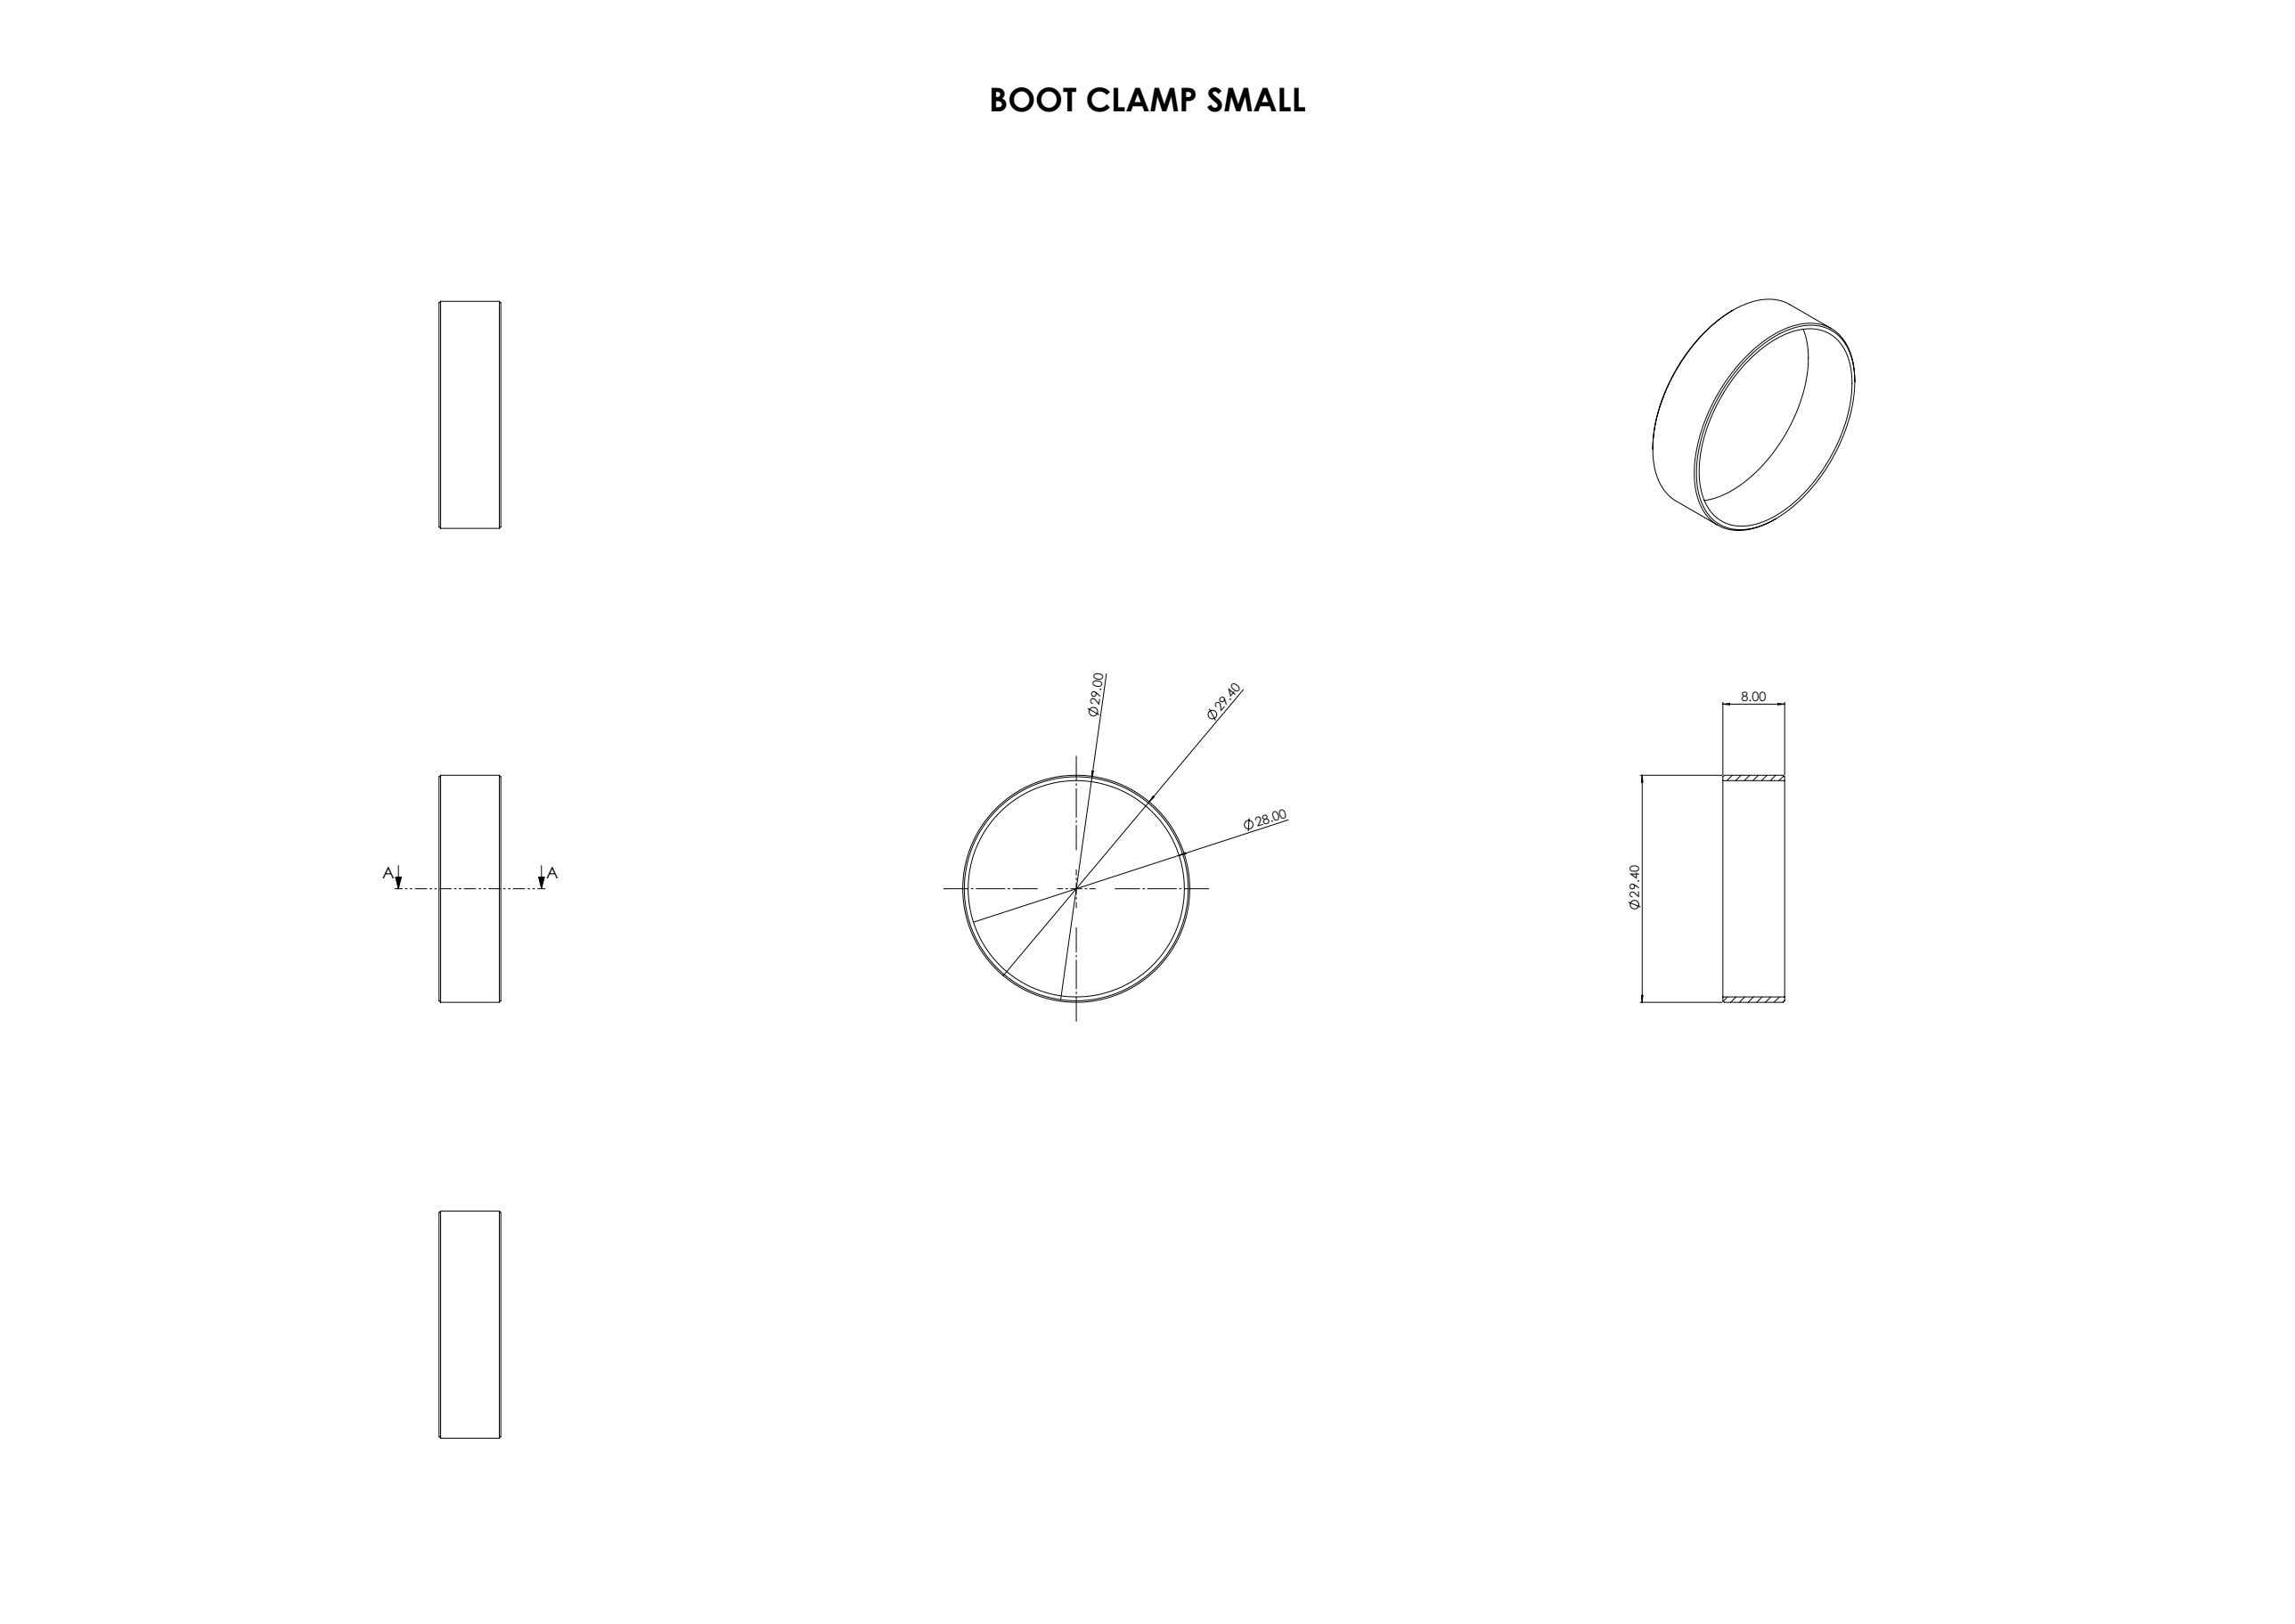
ISO-10303-21;
HEADER;
/* Generated by software containing ST-Developer
 * from STEP Tools, Inc. (www.steptools.com) 
 */

FILE_DESCRIPTION(
/* description */ (''),
/* implementation_level */ '2;1');

FILE_NAME(
/* name */ '09_Boot_Clamp_Small.step',
/* time_stamp */ '2026-10-11T12:57:03-07:00',
/* author */ (''),
/* organization */ (''),
/* preprocessor_version */ 'ST-DEVELOPER v20.2',
/* originating_system */ 'Autodesk Translation Framework v15.15.0.0',
/* authorisation */ '');

FILE_SCHEMA (('AUTOMOTIVE_DESIGN { 1 0 10303 214 3 1 1 }'));
ENDSEC;

DATA;
#10=MECHANICAL_DESIGN_GEOMETRIC_PRESENTATION_REPRESENTATION('',(#264),#90374);
#230=SHAPE_REPRESENTATION_RELATIONSHIP('SRR','None',#90449,#247);
#247=ADVANCED_BREP_SHAPE_REPRESENTATION('',(#281),#90365);
#264=STYLED_ITEM('',(#90673),#281);
#281=MANIFOLD_SOLID_BREP('Body1',#40353);
#691=CONICAL_SURFACE('',#43833,14.6,0.785398163397449);
#692=CONICAL_SURFACE('',#43838,14.6,0.785398163397448);
#1071=FACE_BOUND('',#6255,.T.);
#1072=FACE_BOUND('',#6258,.T.);
#1441=PLANE('',#43840);
#1442=PLANE('',#43844);
#3823=FACE_OUTER_BOUND('',#6251,.T.);
#3824=FACE_OUTER_BOUND('',#6252,.T.);
#3825=FACE_OUTER_BOUND('',#6253,.T.);
#3826=FACE_OUTER_BOUND('',#6254,.T.);
#3827=FACE_OUTER_BOUND('',#6256,.T.);
#3828=FACE_OUTER_BOUND('',#6257,.T.);
#6251=EDGE_LOOP('',(#33331,#33332,#33333,#33334));
#6252=EDGE_LOOP('',(#33335,#33336,#33337,#33338));
#6253=EDGE_LOOP('',(#33339,#33340,#33341,#33342));
#6254=EDGE_LOOP('',(#33343));
#6255=EDGE_LOOP('',(#33344));
#6256=EDGE_LOOP('',(#33345,#33346,#33347,#33348));
#6257=EDGE_LOOP('',(#33349));
#6258=EDGE_LOOP('',(#33350));
#8699=CIRCLE('',#43834,14.7);
#8700=CIRCLE('',#43835,14.5);
#8701=CIRCLE('',#43837,14.7);
#8702=CIRCLE('',#43839,14.5);
#8703=CIRCLE('',#43841,14.);
#8704=CIRCLE('',#43843,14.);
#11851=LINE('',#83003,#14345);
#11852=LINE('',#83008,#14346);
#11853=LINE('',#83012,#14347);
#11854=LINE('',#83018,#14348);
#14345=VECTOR('',#53359,14.6);
#14346=VECTOR('',#53366,14.7);
#14347=VECTOR('',#53371,14.6);
#14348=VECTOR('',#53378,14.);
#17794=VERTEX_POINT('',#83000);
#17795=VERTEX_POINT('',#83002);
#17796=VERTEX_POINT('',#83006);
#17797=VERTEX_POINT('',#83010);
#17798=VERTEX_POINT('',#83014);
#17799=VERTEX_POINT('',#83017);
#23177=EDGE_CURVE('',#17794,#17794,#8699,.T.);
#23178=EDGE_CURVE('',#17794,#17795,#11851,.T.);
#23179=EDGE_CURVE('',#17795,#17795,#8700,.T.);
#23180=EDGE_CURVE('',#17796,#17796,#8701,.T.);
#23181=EDGE_CURVE('',#17796,#17794,#11852,.T.);
#23182=EDGE_CURVE('',#17797,#17797,#8702,.T.);
#23183=EDGE_CURVE('',#17797,#17796,#11853,.T.);
#23184=EDGE_CURVE('',#17798,#17798,#8703,.T.);
#23185=EDGE_CURVE('',#17798,#17799,#11854,.T.);
#23186=EDGE_CURVE('',#17799,#17799,#8704,.T.);
#33331=ORIENTED_EDGE('',*,*,#23177,.F.);
#33332=ORIENTED_EDGE('',*,*,#23178,.T.);
#33333=ORIENTED_EDGE('',*,*,#23179,.T.);
#33334=ORIENTED_EDGE('',*,*,#23178,.F.);
#33335=ORIENTED_EDGE('',*,*,#23180,.F.);
#33336=ORIENTED_EDGE('',*,*,#23181,.T.);
#33337=ORIENTED_EDGE('',*,*,#23177,.T.);
#33338=ORIENTED_EDGE('',*,*,#23181,.F.);
#33339=ORIENTED_EDGE('',*,*,#23182,.F.);
#33340=ORIENTED_EDGE('',*,*,#23183,.T.);
#33341=ORIENTED_EDGE('',*,*,#23180,.T.);
#33342=ORIENTED_EDGE('',*,*,#23183,.F.);
#33343=ORIENTED_EDGE('',*,*,#23182,.T.);
#33344=ORIENTED_EDGE('',*,*,#23184,.F.);
#33345=ORIENTED_EDGE('',*,*,#23184,.T.);
#33346=ORIENTED_EDGE('',*,*,#23185,.T.);
#33347=ORIENTED_EDGE('',*,*,#23186,.F.);
#33348=ORIENTED_EDGE('',*,*,#23185,.F.);
#33349=ORIENTED_EDGE('',*,*,#23179,.F.);
#33350=ORIENTED_EDGE('',*,*,#23186,.T.);
#37776=CYLINDRICAL_SURFACE('',#43836,14.7);
#37777=CYLINDRICAL_SURFACE('',#43842,14.);
#39626=ADVANCED_FACE('',(#3823),#691,.T.);
#39627=ADVANCED_FACE('',(#3824),#37776,.T.);
#39628=ADVANCED_FACE('',(#3825),#692,.T.);
#39629=ADVANCED_FACE('',(#3826,#1071),#1441,.T.);
#39630=ADVANCED_FACE('',(#3827),#37777,.F.);
#39631=ADVANCED_FACE('',(#3828,#1072),#1442,.T.);
#40353=CLOSED_SHELL('',(#39626,#39627,#39628,#39629,#39630,#39631));
#43832=AXIS2_PLACEMENT_3D('',#82998,#53353,#53354);
#43833=AXIS2_PLACEMENT_3D('',#82999,#53355,#53356);
#43834=AXIS2_PLACEMENT_3D('',#83001,#53357,#53358);
#43835=AXIS2_PLACEMENT_3D('',#83004,#53360,#53361);
#43836=AXIS2_PLACEMENT_3D('',#83005,#53362,#53363);
#43837=AXIS2_PLACEMENT_3D('',#83007,#53364,#53365);
#43838=AXIS2_PLACEMENT_3D('',#83009,#53367,#53368);
#43839=AXIS2_PLACEMENT_3D('',#83011,#53369,#53370);
#43840=AXIS2_PLACEMENT_3D('',#83013,#53372,#53373);
#43841=AXIS2_PLACEMENT_3D('',#83015,#53374,#53375);
#43842=AXIS2_PLACEMENT_3D('',#83016,#53376,#53377);
#43843=AXIS2_PLACEMENT_3D('',#83019,#53379,#53380);
#43844=AXIS2_PLACEMENT_3D('',#83020,#53381,#53382);
#53353=DIRECTION('axis',(0.,0.,1.));
#53354=DIRECTION('refdir',(1.,0.,0.));
#53355=DIRECTION('center_axis',(1.,0.,0.));
#53356=DIRECTION('ref_axis',(0.,1.,0.));
#53357=DIRECTION('center_axis',(1.,0.,0.));
#53358=DIRECTION('ref_axis',(0.,0.,-1.));
#53359=DIRECTION('',(-0.707106781186547,0.707106781186548,8.65956056235494E-17));
#53360=DIRECTION('center_axis',(1.,0.,0.));
#53361=DIRECTION('ref_axis',(0.,0.,-1.));
#53362=DIRECTION('center_axis',(1.,0.,0.));
#53363=DIRECTION('ref_axis',(0.,1.,0.));
#53364=DIRECTION('center_axis',(1.,0.,0.));
#53365=DIRECTION('ref_axis',(0.,0.,-1.));
#53366=DIRECTION('',(-1.,0.,0.));
#53367=DIRECTION('center_axis',(-1.,0.,0.));
#53368=DIRECTION('ref_axis',(0.,1.,0.));
#53369=DIRECTION('center_axis',(1.,0.,0.));
#53370=DIRECTION('ref_axis',(0.,0.,-1.));
#53371=DIRECTION('',(-0.707106781186548,-0.707106781186548,-8.65956056235493E-17));
#53372=DIRECTION('center_axis',(1.,0.,0.));
#53373=DIRECTION('ref_axis',(0.,0.,-1.));
#53374=DIRECTION('center_axis',(1.,0.,0.));
#53375=DIRECTION('ref_axis',(0.,0.,-1.));
#53376=DIRECTION('center_axis',(1.,0.,0.));
#53377=DIRECTION('ref_axis',(0.,1.,0.));
#53378=DIRECTION('',(-1.,0.,0.));
#53379=DIRECTION('center_axis',(1.,0.,0.));
#53380=DIRECTION('ref_axis',(0.,0.,-1.));
#53381=DIRECTION('center_axis',(-1.,0.,0.));
#53382=DIRECTION('ref_axis',(0.,0.,1.));
#82998=CARTESIAN_POINT('',(0.,0.,0.));
#82999=CARTESIAN_POINT('Origin',(0.1,0.,0.));
#83000=CARTESIAN_POINT('',(0.2,-14.7,-1.80023079474661E-15));
#83001=CARTESIAN_POINT('Origin',(0.2,0.,0.));
#83002=CARTESIAN_POINT('',(-2.77555756156289E-16,-14.5,-1.77573785876366E-15));
#83003=CARTESIAN_POINT('',(0.1,-14.6,-1.78798432675514E-15));
#83004=CARTESIAN_POINT('Origin',(0.,0.,0.));
#83005=CARTESIAN_POINT('Origin',(4.,0.,0.));
#83006=CARTESIAN_POINT('',(7.8,-14.7,-1.80023079474661E-15));
#83007=CARTESIAN_POINT('Origin',(7.8,0.,0.));
#83008=CARTESIAN_POINT('',(4.,-14.7,-1.80023079474661E-15));
#83009=CARTESIAN_POINT('Origin',(7.9,0.,0.));
#83010=CARTESIAN_POINT('',(8.,-14.5,-1.77573785876366E-15));
#83011=CARTESIAN_POINT('Origin',(8.,0.,0.));
#83012=CARTESIAN_POINT('',(7.9,-14.6,-1.78798432675514E-15));
#83013=CARTESIAN_POINT('Origin',(8.,14.,0.));
#83014=CARTESIAN_POINT('',(8.,-14.,-1.71450551880629E-15));
#83015=CARTESIAN_POINT('Origin',(8.,0.,0.));
#83016=CARTESIAN_POINT('Origin',(4.,0.,0.));
#83017=CARTESIAN_POINT('',(0.,-14.,-1.71450551880629E-15));
#83018=CARTESIAN_POINT('',(4.,-14.,-1.71450551880629E-15));
#83019=CARTESIAN_POINT('Origin',(0.,0.,0.));
#83020=CARTESIAN_POINT('Origin',(0.,14.5,0.));
#90346=UNCERTAINTY_MEASURE_WITH_UNIT(LENGTH_MEASURE(0.01),#90375,
'DISTANCE_ACCURACY_VALUE',
'Maximum model space distance between geometric entities at asserted c
onnectivities');
#90355=UNCERTAINTY_MEASURE_WITH_UNIT(LENGTH_MEASURE(0.01),#90375,
'DISTANCE_ACCURACY_VALUE',
'Maximum model space distance between geometric entities at asserted c
onnectivities');
#90365=(
GEOMETRIC_REPRESENTATION_CONTEXT(3)
GLOBAL_UNCERTAINTY_ASSIGNED_CONTEXT((#90346))
GLOBAL_UNIT_ASSIGNED_CONTEXT((#90375,#90377,#90378))
REPRESENTATION_CONTEXT('','3D')
);
#90374=(
GEOMETRIC_REPRESENTATION_CONTEXT(3)
GLOBAL_UNCERTAINTY_ASSIGNED_CONTEXT((#90355))
GLOBAL_UNIT_ASSIGNED_CONTEXT((#90375,#90377,#90378))
REPRESENTATION_CONTEXT('','3D')
);
#90375=(
LENGTH_UNIT()
NAMED_UNIT(*)
SI_UNIT(.MILLI.,.METRE.)
);
#90377=(
NAMED_UNIT(*)
PLANE_ANGLE_UNIT()
SI_UNIT($,.RADIAN.)
);
#90378=(
NAMED_UNIT(*)
SI_UNIT($,.STERADIAN.)
SOLID_ANGLE_UNIT()
);
#90388=SHAPE_DEFINITION_REPRESENTATION(#90406,#90449);
#90406=PRODUCT_DEFINITION_SHAPE('',$,#90468);
#90449=SHAPE_REPRESENTATION('',(#43832),#90365);
#90458=PRODUCT_DEFINITION_CONTEXT('part definition',#90514,'design');
#90468=PRODUCT_DEFINITION('2026-10-11-12-53-11-210',
'09_Boot_Clamp_Small',#90486,#90458);
#90486=PRODUCT_DEFINITION_FORMATION('',$,#90525);
#90514=APPLICATION_CONTEXT(
'Core Data for Automotive Mechanical Design Process');
#90515=PRODUCT_CONTEXT('part definition',#90514,'mechanical');
#90525=PRODUCT('2026-10-11-12-53-11-210','09_Boot_Clamp_Small',$,(#90515));
#90667=COLOUR_RGB('Light Blue',0.38,0.62,0.78);
#90668=FILL_AREA_STYLE_COLOUR('',#90667);
#90669=FILL_AREA_STYLE('',(#90668));
#90670=SURFACE_STYLE_FILL_AREA(#90669);
#90671=SURFACE_SIDE_STYLE('',(#90670));
#90672=SURFACE_STYLE_USAGE(.BOTH.,#90671);
#90673=PRESENTATION_STYLE_ASSIGNMENT((#90672));
ENDSEC;
END-ISO-10303-21;
